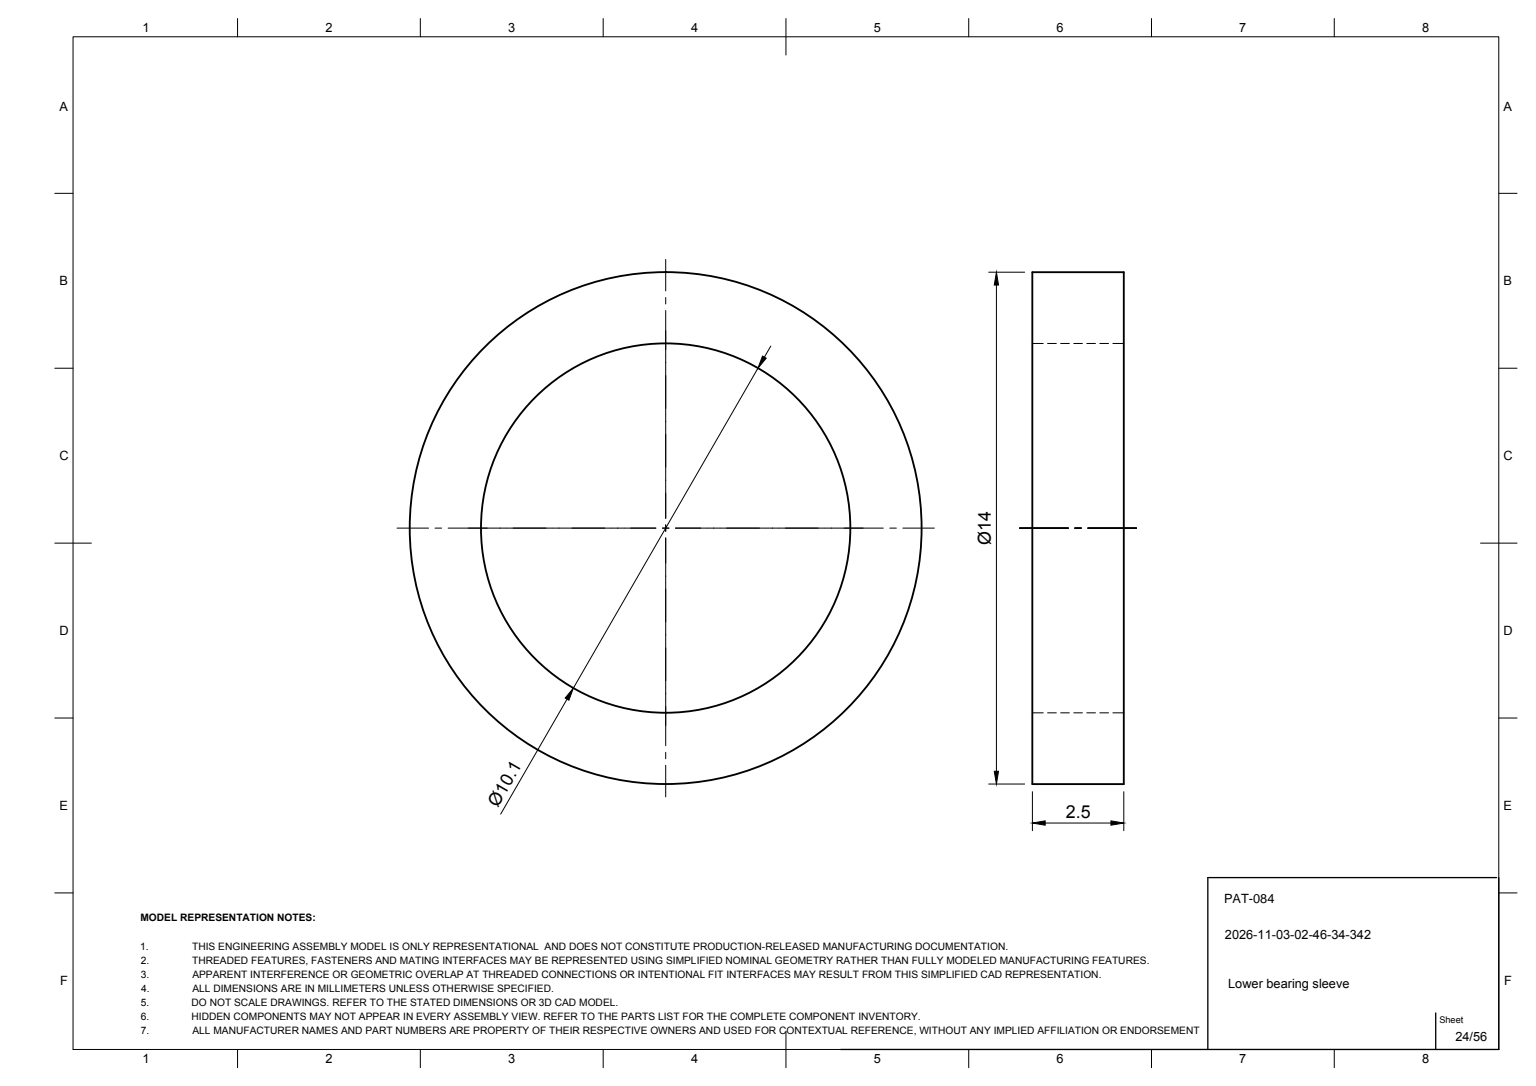
ISO-10303-21;
HEADER;
/* Generated by software containing ST-Developer
 * from STEP Tools, Inc. (www.steptools.com) 
 */

FILE_DESCRIPTION(
/* description */ ('Quick-return (Whitworth) mechanism'),
/* implementation_level */ '2;1');

FILE_NAME(
/* name */ 'Lower bearing sleeve.step',
/* time_stamp */ '2026-10-28T03:25:57-07:00',
/* author */ (''),
/* organization */ (''),
/* preprocessor_version */ 'ST-DEVELOPER v20.2',
/* originating_system */ 'Autodesk Translation Framework v15.17.0.0',
/* authorisation */ '');

FILE_SCHEMA (('AUTOMOTIVE_DESIGN { 1 0 10303 214 3 1 1 }'));
ENDSEC;

DATA;
#10=MECHANICAL_DESIGN_GEOMETRIC_PRESENTATION_REPRESENTATION('',(#513),#14878);
#417=SHAPE_REPRESENTATION_RELATIONSHIP('SRR','None',#15087,#461);
#461=ADVANCED_BREP_SHAPE_REPRESENTATION('',(#565),#14844);
#513=STYLED_ITEM('',(#15406),#565);
#565=MANIFOLD_SOLID_BREP('Body1',#7867);
#709=FACE_BOUND('',#1856,.T.);
#710=FACE_BOUND('',#1858,.T.);
#884=PLANE('',#8893);
#885=PLANE('',#8894);
#1269=FACE_OUTER_BOUND('',#1853,.T.);
#1270=FACE_OUTER_BOUND('',#1854,.T.);
#1271=FACE_OUTER_BOUND('',#1855,.T.);
#1272=FACE_OUTER_BOUND('',#1857,.T.);
#1853=EDGE_LOOP('',(#6214,#6215,#6216,#6217));
#1854=EDGE_LOOP('',(#6218,#6219,#6220,#6221));
#1855=EDGE_LOOP('',(#6222));
#1856=EDGE_LOOP('',(#6223));
#1857=EDGE_LOOP('',(#6224));
#1858=EDGE_LOOP('',(#6225));
#2364=LINE('',#13475,#2887);
#2365=LINE('',#13481,#2888);
#2887=VECTOR('',#10601,0.505);
#2888=VECTOR('',#10608,0.7);
#3472=CIRCLE('',#8888,0.505);
#3473=CIRCLE('',#8889,0.505);
#3474=CIRCLE('',#8891,0.7);
#3475=CIRCLE('',#8892,0.7);
#3959=VERTEX_POINT('',#13472);
#3960=VERTEX_POINT('',#13474);
#3961=VERTEX_POINT('',#13478);
#3962=VERTEX_POINT('',#13480);
#4764=EDGE_CURVE('',#3959,#3959,#3472,.T.);
#4765=EDGE_CURVE('',#3959,#3960,#2364,.T.);
#4766=EDGE_CURVE('',#3960,#3960,#3473,.T.);
#4767=EDGE_CURVE('',#3961,#3961,#3474,.T.);
#4768=EDGE_CURVE('',#3961,#3962,#2365,.T.);
#4769=EDGE_CURVE('',#3962,#3962,#3475,.T.);
#6214=ORIENTED_EDGE('',*,*,#4764,.F.);
#6215=ORIENTED_EDGE('',*,*,#4765,.T.);
#6216=ORIENTED_EDGE('',*,*,#4766,.T.);
#6217=ORIENTED_EDGE('',*,*,#4765,.F.);
#6218=ORIENTED_EDGE('',*,*,#4767,.F.);
#6219=ORIENTED_EDGE('',*,*,#4768,.T.);
#6220=ORIENTED_EDGE('',*,*,#4769,.T.);
#6221=ORIENTED_EDGE('',*,*,#4768,.F.);
#6222=ORIENTED_EDGE('',*,*,#4767,.T.);
#6223=ORIENTED_EDGE('',*,*,#4764,.T.);
#6224=ORIENTED_EDGE('',*,*,#4769,.F.);
#6225=ORIENTED_EDGE('',*,*,#4766,.F.);
#7308=CYLINDRICAL_SURFACE('',#8887,0.505);
#7309=CYLINDRICAL_SURFACE('',#8890,0.7);
#7600=ADVANCED_FACE('',(#1269),#7308,.F.);
#7601=ADVANCED_FACE('',(#1270),#7309,.T.);
#7602=ADVANCED_FACE('',(#1271,#709),#884,.T.);
#7603=ADVANCED_FACE('',(#1272,#710),#885,.F.);
#7867=CLOSED_SHELL('',(#7600,#7601,#7602,#7603));
#8886=AXIS2_PLACEMENT_3D('',#13470,#10595,#10596);
#8887=AXIS2_PLACEMENT_3D('',#13471,#10597,#10598);
#8888=AXIS2_PLACEMENT_3D('',#13473,#10599,#10600);
#8889=AXIS2_PLACEMENT_3D('',#13476,#10602,#10603);
#8890=AXIS2_PLACEMENT_3D('',#13477,#10604,#10605);
#8891=AXIS2_PLACEMENT_3D('',#13479,#10606,#10607);
#8892=AXIS2_PLACEMENT_3D('',#13482,#10609,#10610);
#8893=AXIS2_PLACEMENT_3D('',#13483,#10611,#10612);
#8894=AXIS2_PLACEMENT_3D('',#13484,#10613,#10614);
#10595=DIRECTION('axis',(0.,0.,1.));
#10596=DIRECTION('refdir',(1.,0.,0.));
#10597=DIRECTION('center_axis',(0.,0.,1.));
#10598=DIRECTION('ref_axis',(1.,0.,0.));
#10599=DIRECTION('center_axis',(0.,0.,-1.));
#10600=DIRECTION('ref_axis',(1.,0.,0.));
#10601=DIRECTION('',(0.,0.,-1.));
#10602=DIRECTION('center_axis',(0.,0.,-1.));
#10603=DIRECTION('ref_axis',(1.,0.,0.));
#10604=DIRECTION('center_axis',(0.,0.,1.));
#10605=DIRECTION('ref_axis',(1.,0.,0.));
#10606=DIRECTION('center_axis',(0.,0.,1.));
#10607=DIRECTION('ref_axis',(1.,0.,0.));
#10608=DIRECTION('',(0.,0.,-1.));
#10609=DIRECTION('center_axis',(0.,0.,1.));
#10610=DIRECTION('ref_axis',(1.,0.,0.));
#10611=DIRECTION('center_axis',(0.,0.,1.));
#10612=DIRECTION('ref_axis',(1.,0.,0.));
#10613=DIRECTION('center_axis',(0.,0.,1.));
#10614=DIRECTION('ref_axis',(1.,0.,0.));
#13470=CARTESIAN_POINT('',(0.,0.,0.));
#13471=CARTESIAN_POINT('Origin',(0.,6.,1.8));
#13472=CARTESIAN_POINT('',(-0.505,6.,2.05));
#13473=CARTESIAN_POINT('Origin',(0.,6.,2.05));
#13474=CARTESIAN_POINT('',(-0.505,6.,1.8));
#13475=CARTESIAN_POINT('',(-0.505,6.,1.8));
#13476=CARTESIAN_POINT('Origin',(0.,6.,1.8));
#13477=CARTESIAN_POINT('Origin',(0.,6.,1.8));
#13478=CARTESIAN_POINT('',(-0.7,6.,2.05));
#13479=CARTESIAN_POINT('Origin',(0.,6.,2.05));
#13480=CARTESIAN_POINT('',(-0.7,6.,1.8));
#13481=CARTESIAN_POINT('',(-0.7,6.,1.8));
#13482=CARTESIAN_POINT('Origin',(0.,6.,1.8));
#13483=CARTESIAN_POINT('Origin',(0.,6.,2.05));
#13484=CARTESIAN_POINT('Origin',(0.,6.,1.8));
#14790=UNCERTAINTY_MEASURE_WITH_UNIT(LENGTH_MEASURE(0.001),#14879,
'DISTANCE_ACCURACY_VALUE',
'Maximum model space distance between geometric entities at asserted c
onnectivities');
#14824=UNCERTAINTY_MEASURE_WITH_UNIT(LENGTH_MEASURE(0.001),#14879,
'DISTANCE_ACCURACY_VALUE',
'Maximum model space distance between geometric entities at asserted c
onnectivities');
#14844=(
GEOMETRIC_REPRESENTATION_CONTEXT(3)
GLOBAL_UNCERTAINTY_ASSIGNED_CONTEXT((#14790))
GLOBAL_UNIT_ASSIGNED_CONTEXT((#14879,#14881,#14882))
REPRESENTATION_CONTEXT('','3D')
);
#14878=(
GEOMETRIC_REPRESENTATION_CONTEXT(3)
GLOBAL_UNCERTAINTY_ASSIGNED_CONTEXT((#14824))
GLOBAL_UNIT_ASSIGNED_CONTEXT((#14879,#14881,#14882))
REPRESENTATION_CONTEXT('','3D')
);
#14879=(
LENGTH_UNIT()
NAMED_UNIT(*)
SI_UNIT(.CENTI.,.METRE.)
);
#14881=(
NAMED_UNIT(*)
PLANE_ANGLE_UNIT()
SI_UNIT($,.RADIAN.)
);
#14882=(
NAMED_UNIT(*)
SI_UNIT($,.STERADIAN.)
SOLID_ANGLE_UNIT()
);
#14902=SHAPE_DEFINITION_REPRESENTATION(#14960,#15087);
#14960=PRODUCT_DEFINITION_SHAPE('',$,#15141);
#15087=SHAPE_REPRESENTATION('',(#8886),#14844);
#15121=PRODUCT_DEFINITION_CONTEXT('part definition',#15282,'design');
#15141=PRODUCT_DEFINITION('Lower bearing sleeve','Lower bearing sleeve',
#15194,#15121);
#15194=PRODUCT_DEFINITION_FORMATION('',$,#15303);
#15282=APPLICATION_CONTEXT(
'Core Data for Automotive Mechanical Design Process');
#15283=PRODUCT_CONTEXT('part definition',#15282,'mechanical');
#15303=PRODUCT('Lower bearing sleeve','Lower bearing sleeve',
'Lower bearing sleeve',(#15283));
#15400=COLOUR_RGB('Grey',0.48,0.52,0.57);
#15401=FILL_AREA_STYLE_COLOUR('',#15400);
#15402=FILL_AREA_STYLE('',(#15401));
#15403=SURFACE_STYLE_FILL_AREA(#15402);
#15404=SURFACE_SIDE_STYLE('',(#15403));
#15405=SURFACE_STYLE_USAGE(.BOTH.,#15404);
#15406=PRESENTATION_STYLE_ASSIGNMENT((#15405));
ENDSEC;
END-ISO-10303-21;
